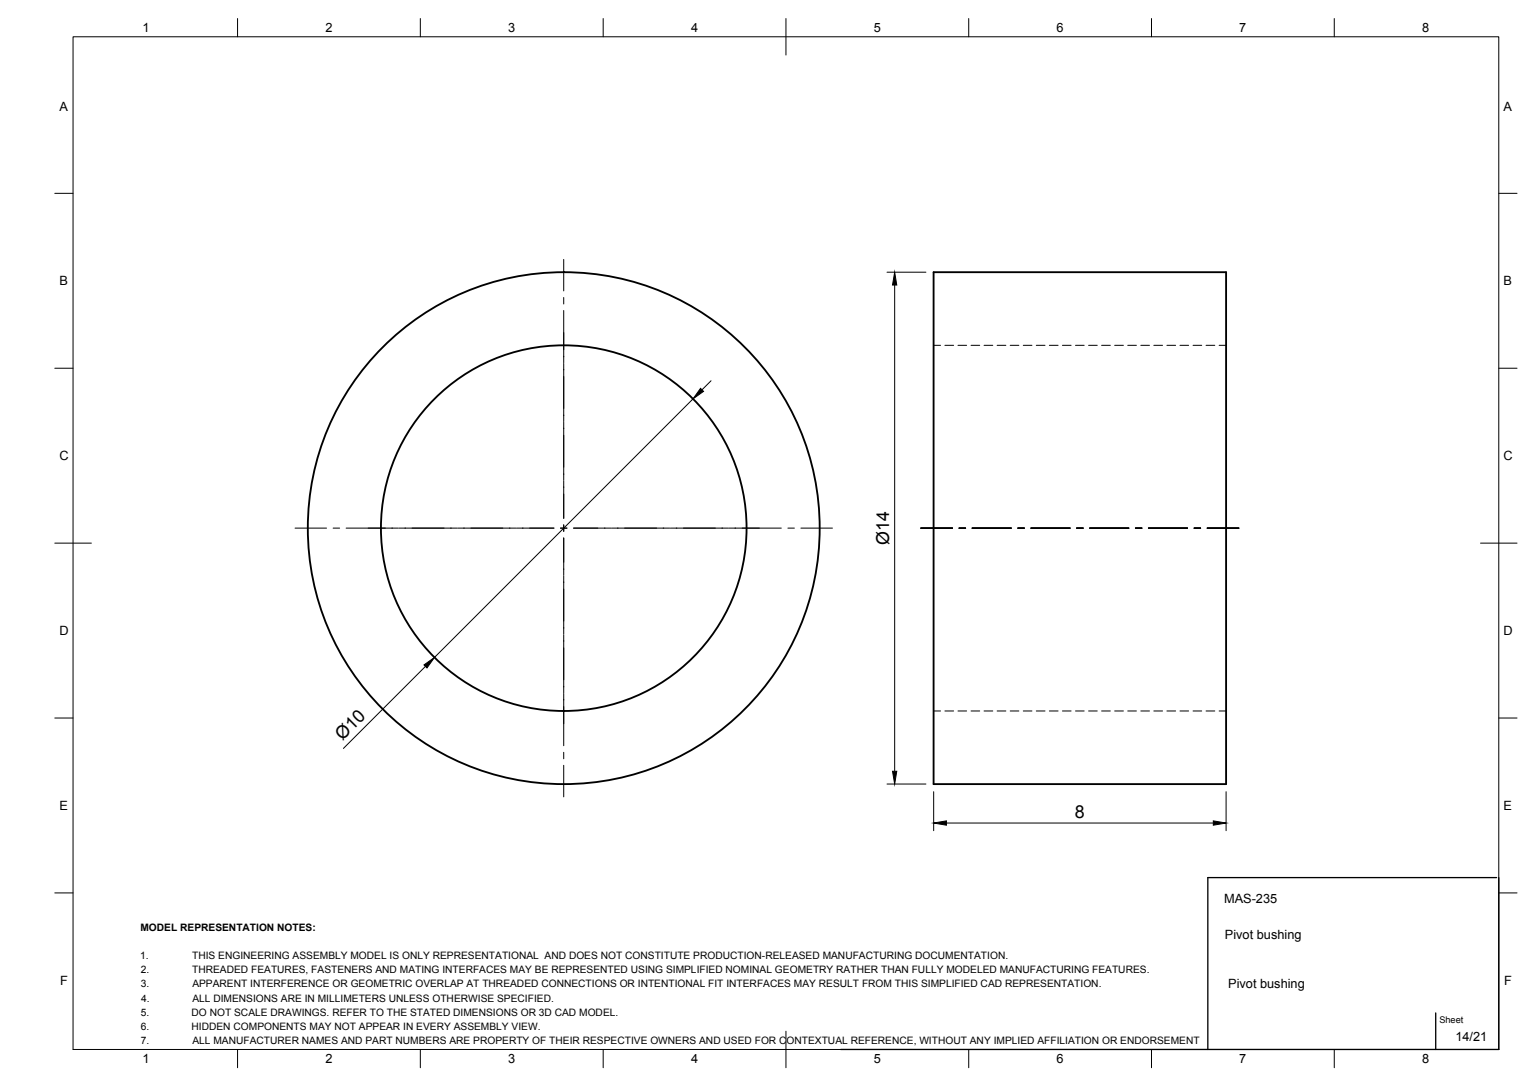
ISO-10303-21;
HEADER;
/* Generated by software containing ST-Developer
 * from STEP Tools, Inc. (www.steptools.com) 
 */

FILE_DESCRIPTION(
/* description */ ('Independent Whitworth quick-return mechanism. Crank radius40, ground-
center spacing80, lever180, connecting rod160, output guide X200. Nomi
nal stroke180 and long/short phase ratio2. Retained guide rods, replac
eable bearing sleeves and captured sliding shoe. No load or production
 rating assigned.'),
/* implementation_level */ '2;1');

FILE_NAME(
/* name */ 'Pivot bushing.step',
/* time_stamp */ '2026-11-09T18:22:56-08:00',
/* author */ (''),
/* organization */ (''),
/* preprocessor_version */ 'ST-DEVELOPER v20.2',
/* originating_system */ 'Autodesk Translation Framework v15.17.0.0',
/* authorisation */ '');

FILE_SCHEMA (('AUTOMOTIVE_DESIGN { 1 0 10303 214 3 1 1 }'));
ENDSEC;

DATA;
#10=MECHANICAL_DESIGN_GEOMETRIC_PRESENTATION_REPRESENTATION('',(#235),#4388);
#195=SHAPE_REPRESENTATION_RELATIONSHIP('SRR','None',#4494,#215);
#215=ADVANCED_BREP_SHAPE_REPRESENTATION('',(#255),#4384);
#235=STYLED_ITEM('',(#4596),#255);
#255=MANIFOLD_SOLID_BREP('Body1',#2340);
#313=FACE_BOUND('',#738,.T.);
#314=FACE_BOUND('',#740,.T.);
#395=PLANE('',#2824);
#396=PLANE('',#2825);
#534=FACE_OUTER_BOUND('',#735,.T.);
#535=FACE_OUTER_BOUND('',#736,.T.);
#536=FACE_OUTER_BOUND('',#737,.T.);
#537=FACE_OUTER_BOUND('',#739,.T.);
#735=EDGE_LOOP('',(#2056,#2057,#2058,#2059));
#736=EDGE_LOOP('',(#2060,#2061,#2062,#2063));
#737=EDGE_LOOP('',(#2064));
#738=EDGE_LOOP('',(#2065));
#739=EDGE_LOOP('',(#2066));
#740=EDGE_LOOP('',(#2067));
#884=LINE('',#4236,#1023);
#885=LINE('',#4242,#1024);
#1023=VECTOR('',#3532,5.);
#1024=VECTOR('',#3539,7.);
#1143=CIRCLE('',#2819,5.);
#1144=CIRCLE('',#2820,5.);
#1145=CIRCLE('',#2822,7.);
#1146=CIRCLE('',#2823,7.);
#1313=VERTEX_POINT('',#4233);
#1314=VERTEX_POINT('',#4235);
#1315=VERTEX_POINT('',#4239);
#1316=VERTEX_POINT('',#4241);
#1564=EDGE_CURVE('',#1313,#1313,#1143,.T.);
#1565=EDGE_CURVE('',#1313,#1314,#884,.T.);
#1566=EDGE_CURVE('',#1314,#1314,#1144,.T.);
#1567=EDGE_CURVE('',#1315,#1315,#1145,.T.);
#1568=EDGE_CURVE('',#1315,#1316,#885,.T.);
#1569=EDGE_CURVE('',#1316,#1316,#1146,.T.);
#2056=ORIENTED_EDGE('',*,*,#1564,.F.);
#2057=ORIENTED_EDGE('',*,*,#1565,.T.);
#2058=ORIENTED_EDGE('',*,*,#1566,.T.);
#2059=ORIENTED_EDGE('',*,*,#1565,.F.);
#2060=ORIENTED_EDGE('',*,*,#1567,.F.);
#2061=ORIENTED_EDGE('',*,*,#1568,.T.);
#2062=ORIENTED_EDGE('',*,*,#1569,.T.);
#2063=ORIENTED_EDGE('',*,*,#1568,.F.);
#2064=ORIENTED_EDGE('',*,*,#1567,.T.);
#2065=ORIENTED_EDGE('',*,*,#1564,.T.);
#2066=ORIENTED_EDGE('',*,*,#1569,.F.);
#2067=ORIENTED_EDGE('',*,*,#1566,.F.);
#2169=CYLINDRICAL_SURFACE('',#2818,5.);
#2170=CYLINDRICAL_SURFACE('',#2821,7.);
#2306=ADVANCED_FACE('',(#534),#2169,.F.);
#2307=ADVANCED_FACE('',(#535),#2170,.T.);
#2308=ADVANCED_FACE('',(#536,#313),#395,.T.);
#2309=ADVANCED_FACE('',(#537,#314),#396,.F.);
#2340=CLOSED_SHELL('',(#2306,#2307,#2308,#2309));
#2817=AXIS2_PLACEMENT_3D('',#4231,#3526,#3527);
#2818=AXIS2_PLACEMENT_3D('',#4232,#3528,#3529);
#2819=AXIS2_PLACEMENT_3D('',#4234,#3530,#3531);
#2820=AXIS2_PLACEMENT_3D('',#4237,#3533,#3534);
#2821=AXIS2_PLACEMENT_3D('',#4238,#3535,#3536);
#2822=AXIS2_PLACEMENT_3D('',#4240,#3537,#3538);
#2823=AXIS2_PLACEMENT_3D('',#4243,#3540,#3541);
#2824=AXIS2_PLACEMENT_3D('',#4244,#3542,#3543);
#2825=AXIS2_PLACEMENT_3D('',#4245,#3544,#3545);
#3526=DIRECTION('axis',(0.,0.,1.));
#3527=DIRECTION('refdir',(1.,0.,0.));
#3528=DIRECTION('center_axis',(0.,0.,1.));
#3529=DIRECTION('ref_axis',(1.,0.,0.));
#3530=DIRECTION('center_axis',(0.,0.,-1.));
#3531=DIRECTION('ref_axis',(1.,0.,0.));
#3532=DIRECTION('',(0.,0.,-1.));
#3533=DIRECTION('center_axis',(0.,0.,-1.));
#3534=DIRECTION('ref_axis',(1.,0.,0.));
#3535=DIRECTION('center_axis',(0.,0.,1.));
#3536=DIRECTION('ref_axis',(1.,0.,0.));
#3537=DIRECTION('center_axis',(0.,0.,1.));
#3538=DIRECTION('ref_axis',(1.,0.,0.));
#3539=DIRECTION('',(0.,0.,-1.));
#3540=DIRECTION('center_axis',(0.,0.,1.));
#3541=DIRECTION('ref_axis',(1.,0.,0.));
#3542=DIRECTION('center_axis',(0.,0.,1.));
#3543=DIRECTION('ref_axis',(1.,0.,0.));
#3544=DIRECTION('center_axis',(0.,0.,1.));
#3545=DIRECTION('ref_axis',(1.,0.,0.));
#4231=CARTESIAN_POINT('',(0.,0.,0.));
#4232=CARTESIAN_POINT('Origin',(0.,0.,0.));
#4233=CARTESIAN_POINT('',(-5.,-6.12323399573677E-16,8.));
#4234=CARTESIAN_POINT('Origin',(0.,0.,8.));
#4235=CARTESIAN_POINT('',(-5.,-6.12323399573677E-16,0.));
#4236=CARTESIAN_POINT('',(-5.,-6.12323399573677E-16,0.));
#4237=CARTESIAN_POINT('Origin',(0.,0.,0.));
#4238=CARTESIAN_POINT('Origin',(0.,0.,0.));
#4239=CARTESIAN_POINT('',(-7.,-8.57252759403147E-16,8.));
#4240=CARTESIAN_POINT('Origin',(0.,0.,8.));
#4241=CARTESIAN_POINT('',(-7.,-8.57252759403147E-16,0.));
#4242=CARTESIAN_POINT('',(-7.,-8.57252759403147E-16,0.));
#4243=CARTESIAN_POINT('Origin',(0.,0.,0.));
#4244=CARTESIAN_POINT('Origin',(0.,0.,8.));
#4245=CARTESIAN_POINT('Origin',(0.,0.,0.));
#4362=UNCERTAINTY_MEASURE_WITH_UNIT(LENGTH_MEASURE(0.01),#4389,
'DISTANCE_ACCURACY_VALUE',
'Maximum model space distance between geometric entities at asserted c
onnectivities');
#4366=UNCERTAINTY_MEASURE_WITH_UNIT(LENGTH_MEASURE(0.01),#4389,
'DISTANCE_ACCURACY_VALUE',
'Maximum model space distance between geometric entities at asserted c
onnectivities');
#4384=(
GEOMETRIC_REPRESENTATION_CONTEXT(3)
GLOBAL_UNCERTAINTY_ASSIGNED_CONTEXT((#4362))
GLOBAL_UNIT_ASSIGNED_CONTEXT((#4389,#4391,#4392))
REPRESENTATION_CONTEXT('','3D')
);
#4388=(
GEOMETRIC_REPRESENTATION_CONTEXT(3)
GLOBAL_UNCERTAINTY_ASSIGNED_CONTEXT((#4366))
GLOBAL_UNIT_ASSIGNED_CONTEXT((#4389,#4391,#4392))
REPRESENTATION_CONTEXT('','3D')
);
#4389=(
LENGTH_UNIT()
NAMED_UNIT(*)
SI_UNIT(.MILLI.,.METRE.)
);
#4391=(
NAMED_UNIT(*)
PLANE_ANGLE_UNIT()
SI_UNIT($,.RADIAN.)
);
#4392=(
NAMED_UNIT(*)
SI_UNIT($,.STERADIAN.)
SOLID_ANGLE_UNIT()
);
#4410=SHAPE_DEFINITION_REPRESENTATION(#4431,#4494);
#4431=PRODUCT_DEFINITION_SHAPE('',$,#4516);
#4494=SHAPE_REPRESENTATION('',(#2817),#4384);
#4498=PRODUCT_DEFINITION_CONTEXT('part definition',#4563,'design');
#4516=PRODUCT_DEFINITION('Pivot bushing','Pivot bushing',#4537,#4498);
#4537=PRODUCT_DEFINITION_FORMATION('',$,#4582);
#4563=APPLICATION_CONTEXT(
'Core Data for Automotive Mechanical Design Process');
#4564=PRODUCT_CONTEXT('part definition',#4563,'mechanical');
#4582=PRODUCT('Pivot bushing','Pivot bushing',$,(#4564));
#4596=PRESENTATION_STYLE_ASSIGNMENT((#4610));
#4610=SURFACE_STYLE_USAGE(.BOTH.,#4624);
#4624=SURFACE_SIDE_STYLE('',(#4638));
#4638=SURFACE_STYLE_FILL_AREA(#4652);
#4652=FILL_AREA_STYLE('Bearing light gray',(#4666));
#4666=FILL_AREA_STYLE_COLOUR('Bearing light gray',#4680);
#4680=COLOUR_RGB('Bearing light gray',0.725490196078431,0.752941176470588,
0.792156862745098);
ENDSEC;
END-ISO-10303-21;
